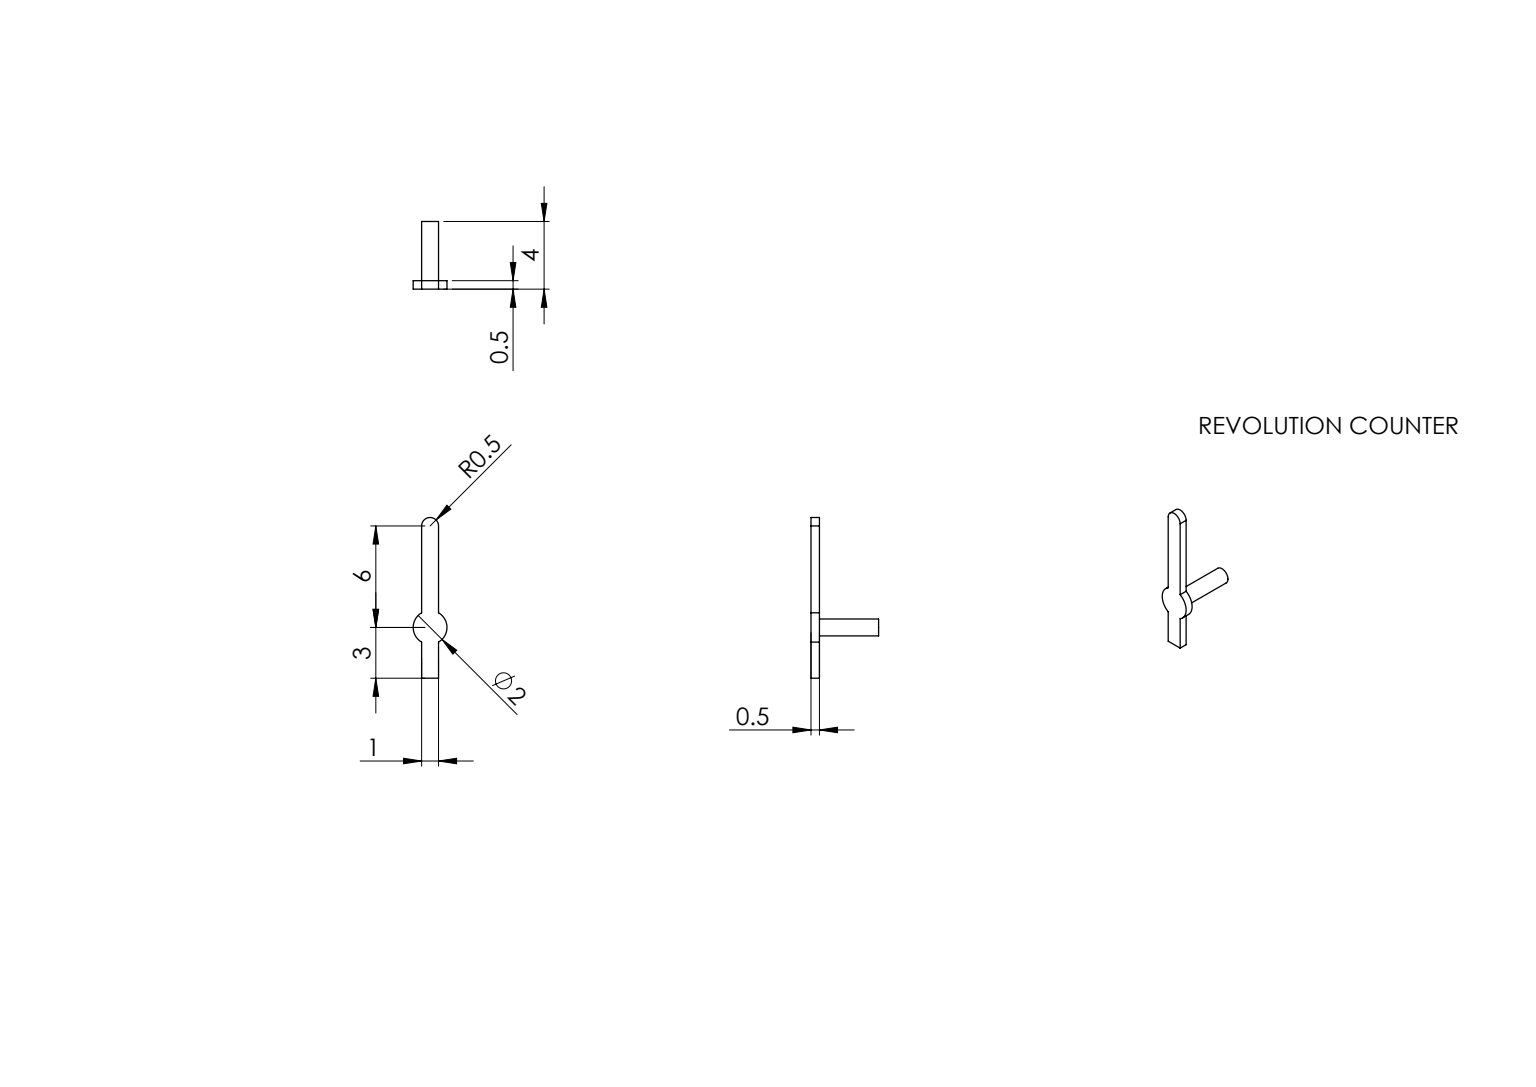
ISO-10303-21;
HEADER;
FILE_DESCRIPTION (('STEP AP214'),
    '1' );
FILE_NAME ('revolution counter.step',
    '2026-10-26T12:50:16',
    ( '' ),
    ( '' ),
    'SwSTEP 2.0',
    'SolidWorks 2026',
    '' );
FILE_SCHEMA (( 'AUTOMOTIVE_DESIGN' ));
ENDSEC;

DATA;
#137=AXIS2_PLACEMENT_3D ( 'NONE', #2400, #6189, #455 ) ;
#284=VERTEX_POINT ( 'NONE', #18909 ) ;
#335=CARTESIAN_POINT ( 'NONE',  ( 0.000000000000000000, 0.000000000000000000, 20.00000000000000000 ) ) ;
#373=CARTESIAN_POINT ( 'NONE',  ( 0.5000000000000001110, 6.123233995736767268E-17, 19.50000000000000000 ) ) ;
#380=VERTEX_POINT ( 'NONE', #21626 ) ;
#455=DIRECTION ( 'NONE',  ( 1.000000000000000000, 0.000000000000000000, 0.000000000000000000 ) ) ;
#566=DIRECTION ( 'NONE',  ( 0.000000000000000000, 0.000000000000000000, 1.000000000000000000 ) ) ;
#582=( GEOMETRIC_REPRESENTATION_CONTEXT ( 3 ) GLOBAL_UNCERTAINTY_ASSIGNED_CONTEXT ( ( #20915 ) ) GLOBAL_UNIT_ASSIGNED_CONTEXT ( ( #19068, #4949, #20517 ) ) REPRESENTATION_CONTEXT ( 'NONE', 'WORKASPACE' ) );
#828=AXIS2_PLACEMENT_3D ( 'NONE', #14567, #3180, #16661 ) ;
#850=AXIS2_PLACEMENT_3D ( 'NONE', #16943, #22823, #13265 ) ;
#918=CARTESIAN_POINT ( 'NONE',  ( 0.5000000000000000000, -2.999999999999999556, 19.50000000000000000 ) ) ;
#963=PLANE ( 'NONE',  #13721 ) ;
#1144=EDGE_CURVE ( 'NONE', #20048, #24513, #24920, .T. ) ;
#1198=DIRECTION ( 'NONE',  ( 1.000000000000000000, 0.000000000000000000, 0.000000000000000000 ) ) ;
#1235=ORIENTED_EDGE ( 'NONE', *, *, #22619, .T. ) ;
#1238=ADVANCED_FACE ( 'NONE', ( #9863 ), #7774, .T. ) ;
#1249=AXIS2_PLACEMENT_3D ( 'NONE', #11596, #19570, #3891 ) ;
#1274=VECTOR ( 'NONE', #23416, 1000.000000000000000 ) ;
#1303=ADVANCED_BREP_SHAPE_REPRESENTATION ( '', ( #5435, #21036 ), #582 ) ;
#1310=AXIS2_PLACEMENT_3D ( 'NONE', #12384, #20350, #10407 ) ;
#1424=FACE_OUTER_BOUND ( 'NONE', #1773, .T. ) ;
#1576=LINE ( 'NONE', #19611, #1274 ) ;
#1773=EDGE_LOOP ( 'NONE', ( #24159, #22801, #5797, #22926 ) ) ;
#1809=EDGE_CURVE ( 'NONE', #2418, #22249, #8902, .T. ) ;
#1853=CARTESIAN_POINT ( 'NONE',  ( -0.5000000000000000000, 6.000000000000000000, 20.00000000000000000 ) ) ;
#2018=DIRECTION ( 'NONE',  ( -0.000000000000000000, -1.000000000000000000, 0.000000000000000000 ) ) ;
#2037=CIRCLE ( 'NONE', #10361, 0.5000000000000000000 ) ;
#2117=ORIENTED_EDGE ( 'NONE', *, *, #6935, .T. ) ;
#2213=ORIENTED_EDGE ( 'NONE', *, *, #1809, .F. ) ;
#2224=( LENGTH_UNIT ( ) NAMED_UNIT ( * ) SI_UNIT ( .MILLI., .METRE. ) );
#2233=AXIS2_PLACEMENT_3D ( 'NONE', #13758, #15729, #7485 ) ;
#2254=VERTEX_POINT ( 'NONE', #17304 ) ;
#2278=EDGE_CURVE ( 'NONE', #11678, #7709, #7918, .T. ) ;
#2363=ORIENTED_EDGE ( 'NONE', *, *, #13575, .T. ) ;
#2369=ORIENTED_EDGE ( 'NONE', *, *, #6160, .F. ) ;
#2400=CARTESIAN_POINT ( 'NONE',  ( 0.000000000000000000, 0.000000000000000000, 19.50000000000000000 ) ) ;
#2418=VERTEX_POINT ( 'NONE', #14656 ) ;
#2611=VECTOR ( 'NONE', #3149, 1000.000000000000000 ) ;
#2661=STYLED_ITEM ( 'NONE', ( #20909 ), #1303 ) ;
#2797=DIRECTION ( 'NONE',  ( -0.000000000000000000, 0.000000000000000000, 1.000000000000000000 ) ) ;
#2884=ORIENTED_EDGE ( 'NONE', *, *, #22262, .T. ) ;
#2904=AXIS2_PLACEMENT_3D ( 'NONE', #9180, #7226, #15209 ) ;
#2905=DIRECTION ( 'NONE',  ( 0.000000000000000000, 0.000000000000000000, 1.000000000000000000 ) ) ;
#2957=AXIS2_PLACEMENT_3D ( 'NONE', #24182, #8117, #20255 ) ;
#2996=( NAMED_UNIT ( * ) SI_UNIT ( $, .STERADIAN. ) SOLID_ANGLE_UNIT ( ) );
#3029=EDGE_CURVE ( 'NONE', #15016, #11472, #8357, .T. ) ;
#3072=STYLED_ITEM('',(#25900),#5435);
#3121=SURFACE_SIDE_STYLE ('',( #22749 ) ) ;
#3126=UNCERTAINTY_MEASURE_WITH_UNIT (LENGTH_MEASURE( 1.000000000000000082E-05 ), #6522, 'distance_accuracy_value', 'NONE');
#3140=ORIENTED_EDGE ( 'NONE', *, *, #3029, .F. ) ;
#3144=ADVANCED_FACE ( 'NONE', ( #15239 ), #5034, .F. ) ;
#3145=ORIENTED_EDGE ( 'NONE', *, *, #21940, .T. ) ;
#3148=EDGE_LOOP ( 'NONE', ( #22343, #13600, #19888, #25002 ) ) ;
#3149=DIRECTION ( 'NONE',  ( -0.000000000000000000, -1.000000000000000000, 0.000000000000000000 ) ) ;
#3180=DIRECTION ( 'NONE',  ( -0.000000000000000000, -0.000000000000000000, -1.000000000000000000 ) ) ;
#3246=DIRECTION ( 'NONE',  ( 0.000000000000000000, 0.000000000000000000, 1.000000000000000000 ) ) ;
#3285=DIRECTION ( 'NONE',  ( 0.000000000000000000, 0.000000000000000000, 1.000000000000000000 ) ) ;
#3847=VECTOR ( 'NONE', #2018, 1000.000000000000000 ) ;
#3891=DIRECTION ( 'NONE',  ( 1.000000000000000000, 0.000000000000000000, 0.000000000000000000 ) ) ;
#3915=MECHANICAL_DESIGN_GEOMETRIC_PRESENTATION_REPRESENTATION('',(#3072),#10585);
#4021=ORIENTED_EDGE ( 'NONE', *, *, #15996, .F. ) ;
#4113=CARTESIAN_POINT ( 'NONE',  ( 0.5000000000000000000, 0.8660254037844387076, 20.00000000000000000 ) ) ;
#4228=ORIENTED_EDGE ( 'NONE', *, *, #21940, .F. ) ;
#4292=CIRCLE ( 'NONE', #21824, 1.000000000000000000 ) ;
#4309=VECTOR ( 'NONE', #5742, 1000.000000000000000 ) ;
#4360=EDGE_CURVE ( 'NONE', #22434, #380, #13096, .T. ) ;
#4373=PLANE ( 'NONE',  #5511 ) ;
#4395=CARTESIAN_POINT ( 'NONE',  ( 0.000000000000000000, 6.000000000000000000, 19.50000000000000000 ) ) ;
#4453=ORIENTED_EDGE ( 'NONE', *, *, #25200, .F. ) ;
#4592=CIRCLE ( 'NONE', #1249, 1.000000000000000000 ) ;
#4632=AXIS2_PLACEMENT_3D ( 'NONE', #23250, #5093, #9512 ) ;
#4709=AXIS2_PLACEMENT_3D ( 'NONE', #21206, #3285, #1198 ) ;
#4716=DIRECTION ( 'NONE',  ( -1.000000000000000000, 0.000000000000000000, 0.000000000000000000 ) ) ;
#4834=DIRECTION ( 'NONE',  ( 0.000000000000000000, 0.000000000000000000, 1.000000000000000000 ) ) ;
#4949=( NAMED_UNIT ( * ) PLANE_ANGLE_UNIT ( ) SI_UNIT ( $, .RADIAN. ) );
#5025=AXIS2_PLACEMENT_3D ( 'NONE', #16249, #566, #16124 ) ;
#5034=PLANE ( 'NONE',  #850 ) ;
#5051=ADVANCED_FACE ( 'NONE', ( #5679 ), #14322, .T. ) ;
#5057=CIRCLE ( 'NONE', #1310, 0.5000000000000001110 ) ;
#5093=DIRECTION ( 'NONE',  ( 0.000000000000000000, 0.000000000000000000, 1.000000000000000000 ) ) ;
#5133=DIRECTION ( 'NONE',  ( 0.000000000000000000, 0.000000000000000000, -1.000000000000000000 ) ) ;
#5179=ORIENTED_EDGE ( 'NONE', *, *, #11117, .T. ) ;
#5204=ORIENTED_EDGE ( 'NONE', *, *, #10339, .T. ) ;
#5292=EDGE_CURVE ( 'NONE', #16864, #284, #17044, .T. ) ;
#5316=ORIENTED_EDGE ( 'NONE', *, *, #22898, .F. ) ;
#5435=MANIFOLD_SOLID_BREP ( 'Extrude-Thin1', #13391 ) ;
#5507=DIRECTION ( 'NONE',  ( 0.000000000000000000, 0.000000000000000000, 1.000000000000000000 ) ) ;
#5511=AXIS2_PLACEMENT_3D ( 'NONE', #22692, #6338, #2797 ) ;
#5585=VERTEX_POINT ( 'NONE', #22475 ) ;
#5669=ORIENTED_EDGE ( 'NONE', *, *, #10339, .F. ) ;
#5679=FACE_OUTER_BOUND ( 'NONE', #25492, .T. ) ;
#5742=DIRECTION ( 'NONE',  ( -0.000000000000000000, -1.000000000000000000, -0.000000000000000000 ) ) ;
#5785=CYLINDRICAL_SURFACE ( 'NONE', #17629, 1.000000000000000000 ) ;
#5787=EDGE_LOOP ( 'NONE', ( #9592, #8354, #12731, #15077 ) ) ;
#5797=ORIENTED_EDGE ( 'NONE', *, *, #15047, .T. ) ;
#5798=ADVANCED_FACE ( 'NONE', ( #14355 ), #10537, .T. ) ;
#5926=DIRECTION ( 'NONE',  ( 1.000000000000000000, 0.000000000000000000, 0.000000000000000000 ) ) ;
#6106=CARTESIAN_POINT ( 'NONE',  ( -0.5000000000000001110, 0.000000000000000000, 20.00000000000000000 ) ) ;
#6124=ORIENTED_EDGE ( 'NONE', *, *, #2278, .T. ) ;
#6160=EDGE_CURVE ( 'NONE', #380, #2254, #22546, .T. ) ;
#6189=DIRECTION ( 'NONE',  ( 0.000000000000000000, 0.000000000000000000, 1.000000000000000000 ) ) ;
#6338=DIRECTION ( 'NONE',  ( -1.000000000000000000, 0.000000000000000000, -0.000000000000000000 ) ) ;
#6515=VERTEX_POINT ( 'NONE', #15857 ) ;
#6522=( LENGTH_UNIT ( ) NAMED_UNIT ( * ) SI_UNIT ( .MILLI., .METRE. ) );
#6662=DIRECTION ( 'NONE',  ( 1.000000000000000000, 0.000000000000000000, 0.000000000000000000 ) ) ;
#6758=CARTESIAN_POINT ( 'NONE',  ( 0.5000000000000000000, -2.999999999999999556, 19.50000000000000000 ) ) ;
#6890=FACE_BOUND ( 'NONE', #24975, .T. ) ;
#6935=EDGE_CURVE ( 'NONE', #18179, #25045, #16534, .T. ) ;
#7002=EDGE_CURVE ( 'NONE', #5585, #2254, #9190, .T. ) ;
#7027=ORIENTED_EDGE ( 'NONE', *, *, #25200, .T. ) ;
#7205=CARTESIAN_POINT ( 'NONE',  ( 0.5000000000000000000, 0.000000000000000000, 20.00000000000000000 ) ) ;
#7226=DIRECTION ( 'NONE',  ( 0.000000000000000000, 0.000000000000000000, 1.000000000000000000 ) ) ;
#7375=ORIENTED_EDGE ( 'NONE', *, *, #12297, .F. ) ;
#7448=ORIENTED_EDGE ( 'NONE', *, *, #6935, .F. ) ;
#7485=DIRECTION ( 'NONE',  ( 1.000000000000000000, 0.000000000000000000, 0.000000000000000000 ) ) ;
#7570=VECTOR ( 'NONE', #24503, 1000.000000000000000 ) ;
#7689=CARTESIAN_POINT ( 'NONE',  ( 0.5000000000000001110, 6.123233995736767268E-17, 16.00000000000000000 ) ) ;
#7709=VERTEX_POINT ( 'NONE', #13877 ) ;
#7747=VECTOR ( 'NONE', #3246, 1000.000000000000000 ) ;
#7762=EDGE_CURVE ( 'NONE', #18701, #11472, #16218, .T. ) ;
#7767=ORIENTED_EDGE ( 'NONE', *, *, #18911, .F. ) ;
#7774=PLANE ( 'NONE',  #10516 ) ;
#7870=LINE ( 'NONE', #12186, #8778 ) ;
#7918=CIRCLE ( 'NONE', #2904, 0.5000000000000001110 ) ;
#8117=DIRECTION ( 'NONE',  ( 0.000000000000000000, 0.000000000000000000, 1.000000000000000000 ) ) ;
#8162=SHAPE_REPRESENTATION ( 'revolution counter', ( #21036 ), #582 ) ;
#8199=EDGE_CURVE ( 'NONE', #20048, #13450, #4292, .T. ) ;
#8223=ORIENTED_EDGE ( 'NONE', *, *, #18466, .T. ) ;
#8354=ORIENTED_EDGE ( 'NONE', *, *, #19672, .F. ) ;
#8357=CIRCLE ( 'NONE', #22561, 1.000000000000000000 ) ;
#8372=DIRECTION ( 'NONE',  ( -0.000000000000000000, -0.000000000000000000, -1.000000000000000000 ) ) ;
#8398=PRODUCT_DEFINITION_SHAPE ( 'NONE', 'NONE',  #22284 ) ;
#8450=EDGE_CURVE ( 'NONE', #284, #9659, #13897, .T. ) ;
#8469=LINE ( 'NONE', #6758, #13830 ) ;
#8479=LINE ( 'NONE', #16582, #16675 ) ;
#8629=DIRECTION ( 'NONE',  ( 0.000000000000000000, 0.000000000000000000, 1.000000000000000000 ) ) ;
#8679=FACE_OUTER_BOUND ( 'NONE', #13542, .T. ) ;
#8778=VECTOR ( 'NONE', #9960, 1000.000000000000000 ) ;
#8902=LINE ( 'NONE', #13203, #7747 ) ;
#8973=PRODUCT_DEFINITION_FORMATION_WITH_SPECIFIED_SOURCE ( 'ANY', '', #18425, .NOT_KNOWN. ) ;
#9120=AXIS2_PLACEMENT_3D ( 'NONE', #16101, #12416, #6662 ) ;
#9129=DIRECTION ( 'NONE',  ( -1.000000000000000000, 0.000000000000000000, 0.000000000000000000 ) ) ;
#9180=CARTESIAN_POINT ( 'NONE',  ( 0.000000000000000000, 0.000000000000000000, 19.50000000000000000 ) ) ;
#9190=LINE ( 'NONE', #21485, #11772 ) ;
#9272=CYLINDRICAL_SURFACE ( 'NONE', #18007, 0.5000000000000001110 ) ;
#9488=CARTESIAN_POINT ( 'NONE',  ( 0.000000000000000000, 0.000000000000000000, 16.00000000000000000 ) ) ;
#9512=DIRECTION ( 'NONE',  ( 1.000000000000000000, 0.000000000000000000, 0.000000000000000000 ) ) ;
#9514=AXIS2_PLACEMENT_3D ( 'NONE', #16606, #20259, #4834 ) ;
#9540=AXIS2_PLACEMENT_3D ( 'NONE', #15202, #19367, #5133 ) ;
#9568=ORIENTED_EDGE ( 'NONE', *, *, #11117, .F. ) ;
#9592=ORIENTED_EDGE ( 'NONE', *, *, #6160, .T. ) ;
#9604=DIRECTION ( 'NONE',  ( -1.000000000000000000, 0.000000000000000000, 0.000000000000000000 ) ) ;
#9659=VERTEX_POINT ( 'NONE', #23698 ) ;
#9730=EDGE_LOOP ( 'NONE', ( #21499, #20363, #15304, #20579 ) ) ;
#9842=PRODUCT_CONTEXT ( 'NONE', #17136, 'mechanical' ) ;
#9863=FACE_OUTER_BOUND ( 'NONE', #15185, .T. ) ;
#9930=CARTESIAN_POINT ( 'NONE',  ( 1.000000000000000000, 0.000000000000000000, 19.50000000000000000 ) ) ;
#9960=DIRECTION ( 'NONE',  ( 0.000000000000000000, 0.000000000000000000, 1.000000000000000000 ) ) ;
#10107=VECTOR ( 'NONE', #16356, 1000.000000000000000 ) ;
#10233=ORIENTED_EDGE ( 'NONE', *, *, #25420, .T. ) ;
#10248=FACE_OUTER_BOUND ( 'NONE', #14469, .T. ) ;
#10327=VERTEX_POINT ( 'NONE', #7689 ) ;
#10339=EDGE_CURVE ( 'NONE', #7709, #6515, #24026, .T. ) ;
#10361=AXIS2_PLACEMENT_3D ( 'NONE', #20848, #22818, #19240 ) ;
#10370=CARTESIAN_POINT ( 'NONE',  ( -0.5000000000000000000, -2.999999999999999556, 19.50000000000000000 ) ) ;
#10407=DIRECTION ( 'NONE',  ( 1.000000000000000000, 0.000000000000000000, 0.000000000000000000 ) ) ;
#10468=EDGE_CURVE ( 'NONE', #24513, #380, #8469, .T. ) ;
#10478=VECTOR ( 'NONE', #21674, 1000.000000000000000 ) ;
#10507=CARTESIAN_POINT ( 'NONE',  ( 0.5000000000000000000, -2.999999999999999556, 20.00000000000000000 ) ) ;
#10516=AXIS2_PLACEMENT_3D ( 'NONE', #17846, #9604, #15887 ) ;
#10537=CYLINDRICAL_SURFACE ( 'NONE', #18131, 0.5000000000000000000 ) ;
#10585=( GEOMETRIC_REPRESENTATION_CONTEXT ( 3 ) GLOBAL_UNCERTAINTY_ASSIGNED_CONTEXT ( ( #13074 ) ) GLOBAL_UNIT_ASSIGNED_CONTEXT ( ( #2224, #24314, #21702 ) ) REPRESENTATION_CONTEXT ( 'NONE', 'WORKASPACE' ) );
#10595=ORIENTED_EDGE ( 'NONE', *, *, #12297, .T. ) ;
#10683=ORIENTED_EDGE ( 'NONE', *, *, #18911, .T. ) ;
#10754=DIRECTION ( 'NONE',  ( 0.000000000000000000, 1.000000000000000000, 0.000000000000000000 ) ) ;
#10825=FILL_AREA_STYLE ('',( #22618 ) ) ;
#10846=ORIENTED_EDGE ( 'NONE', *, *, #4360, .F. ) ;
#10919=DIRECTION ( 'NONE',  ( -0.000000000000000000, -1.000000000000000000, 0.000000000000000000 ) ) ;
#11017=DIRECTION ( 'NONE',  ( -1.000000000000000000, 0.000000000000000000, -0.000000000000000000 ) ) ;
#11075=LINE ( 'NONE', #15270, #14617 ) ;
#11117=EDGE_CURVE ( 'NONE', #6515, #10327, #5057, .T. ) ;
#11124=LINE ( 'NONE', #9930, #10107 ) ;
#11140=DIRECTION ( 'NONE',  ( -0.000000000000000000, -1.000000000000000000, 0.000000000000000000 ) ) ;
#11159=CARTESIAN_POINT ( 'NONE',  ( 0.5000000000000000000, -0.8660254037844387076, 19.50000000000000000 ) ) ;
#11174=SHAPE_DEFINITION_REPRESENTATION ( #8398, #8162 ) ;
#11212=CYLINDRICAL_SURFACE ( 'NONE', #4632, 1.000000000000000000 ) ;
#11272=EDGE_CURVE ( 'NONE', #10327, #6515, #22168, .T. ) ;
#11296=DIRECTION ( 'NONE',  ( 1.000000000000000000, 0.000000000000000000, 0.000000000000000000 ) ) ;
#11455=DIRECTION ( 'NONE',  ( 0.000000000000000000, 0.000000000000000000, 1.000000000000000000 ) ) ;
#11472=VERTEX_POINT ( 'NONE', #4113 ) ;
#11524=VERTEX_POINT ( 'NONE', #10370 ) ;
#11596=CARTESIAN_POINT ( 'NONE',  ( 0.000000000000000000, 0.000000000000000000, 20.00000000000000000 ) ) ;
#11678=VERTEX_POINT ( 'NONE', #373 ) ;
#11761=ORIENTED_EDGE ( 'NONE', *, *, #11272, .T. ) ;
#11772=VECTOR ( 'NONE', #11140, 1000.000000000000000 ) ;
#11798=VECTOR ( 'NONE', #8629, 1000.000000000000000 ) ;
#12013=PLANE ( 'NONE',  #2957 ) ;
#12140=ORIENTED_EDGE ( 'NONE', *, *, #7002, .T. ) ;
#12178=VECTOR ( 'NONE', #18737, 1000.000000000000000 ) ;
#12186=CARTESIAN_POINT ( 'NONE',  ( -0.5000000000000000000, 6.000000000000000000, 19.50000000000000000 ) ) ;
#12256=CARTESIAN_POINT ( 'NONE',  ( 1.000000000000000000, 0.000000000000000000, 20.00000000000000000 ) ) ;
#12293=PLANE ( 'NONE',  #9514 ) ;
#12296=LINE ( 'NONE', #20001, #23727 ) ;
#12297=EDGE_CURVE ( 'NONE', #13450, #15016, #11124, .T. ) ;
#12384=CARTESIAN_POINT ( 'NONE',  ( 0.000000000000000000, 0.000000000000000000, 16.00000000000000000 ) ) ;
#12416=DIRECTION ( 'NONE',  ( 0.000000000000000000, 0.000000000000000000, 1.000000000000000000 ) ) ;
#12449=ORIENTED_EDGE ( 'NONE', *, *, #5292, .T. ) ;
#12497=DIRECTION ( 'NONE',  ( 0.000000000000000000, 0.000000000000000000, 1.000000000000000000 ) ) ;
#12680=SHAPE_REPRESENTATION_RELATIONSHIP ( 'NONE' , 'NONE' ,  #8162, #1303 ) ;
#12731=ORIENTED_EDGE ( 'NONE', *, *, #18466, .F. ) ;
#12735=CARTESIAN_POINT ( 'NONE',  ( -0.5000000000000000000, 0.000000000000000000, 20.00000000000000000 ) ) ;
#12825=EDGE_CURVE ( 'NONE', #22434, #20048, #21935, .T. ) ;
#12826=EDGE_LOOP ( 'NONE', ( #7767, #2213, #1235, #3145 ) ) ;
#12850=DIRECTION ( 'NONE',  ( -0.000000000000000000, 0.000000000000000000, 1.000000000000000000 ) ) ;
#12863=VECTOR ( 'NONE', #4716, 1000.000000000000000 ) ;
#12930=SURFACE_STYLE_USAGE ( .BOTH. , #3121 ) ;
#12988=CARTESIAN_POINT ( 'NONE',  ( 0.5000000000000000000, 0.000000000000000000, 19.50000000000000000 ) ) ;
#13074=UNCERTAINTY_MEASURE_WITH_UNIT (LENGTH_MEASURE( 1.000000000000000082E-05 ), #2224, 'distance_accuracy_value', 'NONE');
#13096=LINE ( 'NONE', #7205, #2611 ) ;
#13127=CARTESIAN_POINT ( 'NONE',  ( -0.5000000000000000000, 0.000000000000000000, 19.50000000000000000 ) ) ;
#13203=CARTESIAN_POINT ( 'NONE',  ( 0.5000000000000000000, 6.000000000000000000, 19.50000000000000000 ) ) ;
#13223=DIRECTION ( 'NONE',  ( 1.000000000000000000, 0.000000000000000000, 0.000000000000000000 ) ) ;
#13256=LINE ( 'NONE', #15347, #16667 ) ;
#13265=DIRECTION ( 'NONE',  ( 1.000000000000000000, 0.000000000000000000, -0.000000000000000000 ) ) ;
#13353=CARTESIAN_POINT ( 'NONE',  ( 0.000000000000000000, 0.000000000000000000, 0.000000000000000000 ) ) ;
#13391=CLOSED_SHELL ( 'NONE', ( #23377, #5051, #24362, #21588, #23018, #3144, #24892, #1238, #5798, #18036, #23325, #24282, #20502, #18328 ) ) ;
#13450=VERTEX_POINT ( 'NONE', #23045 ) ;
#13542=EDGE_LOOP ( 'NONE', ( #4021, #18849, #5204, #5179 ) ) ;
#13575=EDGE_CURVE ( 'NONE', #13450, #18701, #23381, .T. ) ;
#13600=ORIENTED_EDGE ( 'NONE', *, *, #22898, .T. ) ;
#13694=CARTESIAN_POINT ( 'NONE',  ( 0.5000000000000000000, 6.000000000000000000, 20.00000000000000000 ) ) ;
#13721=AXIS2_PLACEMENT_3D ( 'NONE', #12988, #11017, #12850 ) ;
#13758=CARTESIAN_POINT ( 'NONE',  ( 0.000000000000000000, 0.000000000000000000, 20.00000000000000000 ) ) ;
#13830=VECTOR ( 'NONE', #14743, 1000.000000000000000 ) ;
#13877=CARTESIAN_POINT ( 'NONE',  ( -0.5000000000000001110, 0.000000000000000000, 19.50000000000000000 ) ) ;
#13897=CIRCLE ( 'NONE', #4709, 1.000000000000000000 ) ;
#14207=AXIS2_PLACEMENT_3D ( 'NONE', #23673, #5507, #25512 ) ;
#14322=CYLINDRICAL_SURFACE ( 'NONE', #137, 1.000000000000000000 ) ;
#14354=MECHANICAL_DESIGN_GEOMETRIC_PRESENTATION_REPRESENTATION('',(#2661),#20630);
#14355=FACE_OUTER_BOUND ( 'NONE', #12826, .T. ) ;
#14469=EDGE_LOOP ( 'NONE', ( #25385, #23977, #7027, #21240 ) ) ;
#14567=CARTESIAN_POINT ( 'NONE',  ( 0.000000000000000000, 0.000000000000000000, 20.00000000000000000 ) ) ;
#14593=CARTESIAN_POINT ( 'NONE',  ( -0.5000000000000000000, 0.8660254037844387076, 20.00000000000000000 ) ) ;
#14617=VECTOR ( 'NONE', #16977, 1000.000000000000000 ) ;
#14638=( NAMED_UNIT ( * ) PLANE_ANGLE_UNIT ( ) SI_UNIT ( $, .RADIAN. ) );
#14646=LINE ( 'NONE', #22628, #12863 ) ;
#14656=CARTESIAN_POINT ( 'NONE',  ( 0.5000000000000000000, 6.000000000000000000, 19.50000000000000000 ) ) ;
#14689=CARTESIAN_POINT ( 'NONE',  ( 0.000000000000000000, 0.000000000000000000, 19.50000000000000000 ) ) ;
#14743=DIRECTION ( 'NONE',  ( 0.000000000000000000, 0.000000000000000000, 1.000000000000000000 ) ) ;
#14748=CARTESIAN_POINT ( 'NONE',  ( 0.000000000000000000, 0.000000000000000000, 19.50000000000000000 ) ) ;
#14837=CYLINDRICAL_SURFACE ( 'NONE', #828, 0.5000000000000001110 ) ;
#14873=PLANE ( 'NONE',  #17226 ) ;
#14945=FACE_OUTER_BOUND ( 'NONE', #9730, .T. ) ;
#15016=VERTEX_POINT ( 'NONE', #12256 ) ;
#15047=EDGE_CURVE ( 'NONE', #25045, #284, #13256, .T. ) ;
#15077=ORIENTED_EDGE ( 'NONE', *, *, #10468, .T. ) ;
#15168=FACE_OUTER_BOUND ( 'NONE', #24517, .T. ) ;
#15185=EDGE_LOOP ( 'NONE', ( #22569, #7448, #4228, #12449 ) ) ;
#15202=CARTESIAN_POINT ( 'NONE',  ( 0.5000000000000000000, 0.000000000000000000, 19.50000000000000000 ) ) ;
#15209=DIRECTION ( 'NONE',  ( 1.000000000000000000, 0.000000000000000000, 0.000000000000000000 ) ) ;
#15239=FACE_OUTER_BOUND ( 'NONE', #19737, .T. ) ;
#15270=CARTESIAN_POINT ( 'NONE',  ( -0.5000000000000000000, -0.8660254037844387076, 19.50000000000000000 ) ) ;
#15304=ORIENTED_EDGE ( 'NONE', *, *, #10468, .F. ) ;
#15347=CARTESIAN_POINT ( 'NONE',  ( -0.5000000000000000000, 0.8660254037844387076, 19.50000000000000000 ) ) ;
#15703=DIRECTION ( 'NONE',  ( 0.000000000000000000, 0.000000000000000000, 1.000000000000000000 ) ) ;
#15729=DIRECTION ( 'NONE',  ( 0.000000000000000000, 0.000000000000000000, 1.000000000000000000 ) ) ;
#15857=CARTESIAN_POINT ( 'NONE',  ( -0.5000000000000001110, 0.000000000000000000, 16.00000000000000000 ) ) ;
#15887=DIRECTION ( 'NONE',  ( 0.000000000000000000, 0.000000000000000000, 1.000000000000000000 ) ) ;
#15925=AXIS2_PLACEMENT_3D ( 'NONE', #9488, #11455, #21265 ) ;
#15926=EDGE_CURVE ( 'NONE', #7709, #11678, #19974, .T. ) ;
#15996=EDGE_CURVE ( 'NONE', #11678, #10327, #12296, .T. ) ;
#16024=CARTESIAN_POINT ( 'NONE',  ( -0.5000000000000000000, 0.000000000000000000, 19.50000000000000000 ) ) ;
#16101=CARTESIAN_POINT ( 'NONE',  ( 0.000000000000000000, 0.000000000000000000, 19.50000000000000000 ) ) ;
#16124=DIRECTION ( 'NONE',  ( 1.000000000000000000, 0.000000000000000000, 0.000000000000000000 ) ) ;
#16218=LINE ( 'NONE', #20380, #11798 ) ;
#16249=CARTESIAN_POINT ( 'NONE',  ( 0.000000000000000000, 6.000000000000000000, 19.50000000000000000 ) ) ;
#16295=DIRECTION ( 'NONE',  ( 0.000000000000000000, 0.000000000000000000, 1.000000000000000000 ) ) ;
#16356=DIRECTION ( 'NONE',  ( 0.000000000000000000, 0.000000000000000000, 1.000000000000000000 ) ) ;
#16534=LINE ( 'NONE', #12735, #12178 ) ;
#16582=CARTESIAN_POINT ( 'NONE',  ( -0.5000000000000000000, -2.999999999999999556, 19.50000000000000000 ) ) ;
#16606=CARTESIAN_POINT ( 'NONE',  ( 0.5000000000000000000, -2.999999999999999556, 19.50000000000000000 ) ) ;
#16661=DIRECTION ( 'NONE',  ( -1.000000000000000000, 0.000000000000000000, 0.000000000000000000 ) ) ;
#16667=VECTOR ( 'NONE', #21107, 1000.000000000000000 ) ;
#16675=VECTOR ( 'NONE', #18665, 1000.000000000000000 ) ;
#16703=FACE_OUTER_BOUND ( 'NONE', #21184, .T. ) ;
#16799=APPLICATION_CONTEXT ( 'automotive_design' ) ;
#16864=VERTEX_POINT ( 'NONE', #20322 ) ;
#16943=CARTESIAN_POINT ( 'NONE',  ( 0.000000000000000000, 0.000000000000000000, 16.00000000000000000 ) ) ;
#16977=DIRECTION ( 'NONE',  ( -0.000000000000000000, -0.000000000000000000, -1.000000000000000000 ) ) ;
#16995=PRODUCT_DEFINITION_CONTEXT ( 'detailed design', #16799, 'design' ) ;
#17044=LINE ( 'NONE', #13127, #4309 ) ;
#17136=APPLICATION_CONTEXT ( 'automotive_design' ) ;
#17226=AXIS2_PLACEMENT_3D ( 'NONE', #14748, #20752, #20625 ) ;
#17239=ORIENTED_EDGE ( 'NONE', *, *, #8199, .F. ) ;
#17304=CARTESIAN_POINT ( 'NONE',  ( -0.5000000000000000000, -2.999999999999999556, 20.00000000000000000 ) ) ;
#17629=AXIS2_PLACEMENT_3D ( 'NONE', #22004, #23973, #5926 ) ;
#17634=CARTESIAN_POINT ( 'NONE',  ( 0.000000000000000000, 0.000000000000000000, 20.00000000000000000 ) ) ;
#17729=EDGE_CURVE ( 'NONE', #5585, #9659, #11075, .T. ) ;
#17809=ORIENTED_EDGE ( 'NONE', *, *, #2278, .F. ) ;
#17846=CARTESIAN_POINT ( 'NONE',  ( -0.5000000000000000000, 0.000000000000000000, 19.50000000000000000 ) ) ;
#18007=AXIS2_PLACEMENT_3D ( 'NONE', #17634, #19573, #9129 ) ;
#18036=ADVANCED_FACE ( 'NONE', ( #18987 ), #23287, .T. ) ;
#18065=VECTOR ( 'NONE', #10919, 1000.000000000000000 ) ;
#18123=LINE ( 'NONE', #16024, #3847 ) ;
#18131=AXIS2_PLACEMENT_3D ( 'NONE', #4395, #12497, #24527 ) ;
#18179=VERTEX_POINT ( 'NONE', #1853 ) ;
#18224=ORIENTED_EDGE ( 'NONE', *, *, #7762, .T. ) ;
#18328=ADVANCED_FACE ( 'NONE', ( #20379 ), #12293, .F. ) ;
#18425=PRODUCT ( 'revolution counter', 'revolution counter', '', ( #9842 ) ) ;
#18466=EDGE_CURVE ( 'NONE', #24513, #11524, #14646, .T. ) ;
#18665=DIRECTION ( 'NONE',  ( 0.000000000000000000, 0.000000000000000000, 1.000000000000000000 ) ) ;
#18701=VERTEX_POINT ( 'NONE', #21551 ) ;
#18737=DIRECTION ( 'NONE',  ( -0.000000000000000000, -1.000000000000000000, -0.000000000000000000 ) ) ;
#18849=ORIENTED_EDGE ( 'NONE', *, *, #15926, .F. ) ;
#18909=CARTESIAN_POINT ( 'NONE',  ( -0.5000000000000000000, 0.8660254037844387076, 19.50000000000000000 ) ) ;
#18911=EDGE_CURVE ( 'NONE', #22249, #18179, #2037, .T. ) ;
#18987=FACE_OUTER_BOUND ( 'NONE', #3148, .T. ) ;
#18997=ORIENTED_EDGE ( 'NONE', *, *, #5292, .F. ) ;
#19068=( LENGTH_UNIT ( ) NAMED_UNIT ( * ) SI_UNIT ( .MILLI., .METRE. ) );
#19087=ORIENTED_EDGE ( 'NONE', *, *, #15996, .T. ) ;
#19240=DIRECTION ( 'NONE',  ( 1.000000000000000000, 0.000000000000000000, 0.000000000000000000 ) ) ;
#19367=DIRECTION ( 'NONE',  ( 1.000000000000000000, 0.000000000000000000, 0.000000000000000000 ) ) ;
#19380=ORIENTED_EDGE ( 'NONE', *, *, #22619, .F. ) ;
#19570=DIRECTION ( 'NONE',  ( 0.000000000000000000, 0.000000000000000000, 1.000000000000000000 ) ) ;
#19573=DIRECTION ( 'NONE',  ( -0.000000000000000000, -0.000000000000000000, -1.000000000000000000 ) ) ;
#19611=CARTESIAN_POINT ( 'NONE',  ( 0.5000000000000000000, 0.000000000000000000, 19.50000000000000000 ) ) ;
#19672=EDGE_CURVE ( 'NONE', #11524, #2254, #8479, .T. ) ;
#19737=EDGE_LOOP ( 'NONE', ( #9568, #24171 ) ) ;
#19888=ORIENTED_EDGE ( 'NONE', *, *, #1809, .T. ) ;
#19974=CIRCLE ( 'NONE', #9120, 0.5000000000000001110 ) ;
#20001=CARTESIAN_POINT ( 'NONE',  ( 0.5000000000000001110, 6.123233995736767268E-17, 20.00000000000000000 ) ) ;
#20048=VERTEX_POINT ( 'NONE', #11159 ) ;
#20082=ORIENTED_EDGE ( 'NONE', *, *, #25288, .T. ) ;
#20092=CARTESIAN_POINT ( 'NONE',  ( 0.5000000000000000000, -0.8660254037844387076, 19.50000000000000000 ) ) ;
#20185=CARTESIAN_POINT ( 'NONE',  ( 0.5000000000000000000, 0.000000000000000000, 20.00000000000000000 ) ) ;
#20255=DIRECTION ( 'NONE',  ( 1.000000000000000000, 0.000000000000000000, -0.000000000000000000 ) ) ;
#20259=DIRECTION ( 'NONE',  ( 0.000000000000000000, 1.000000000000000000, -0.000000000000000000 ) ) ;
#20299=ORIENTED_EDGE ( 'NONE', *, *, #8450, .F. ) ;
#20322=CARTESIAN_POINT ( 'NONE',  ( -0.5000000000000000000, 6.000000000000000000, 19.50000000000000000 ) ) ;
#20350=DIRECTION ( 'NONE',  ( 0.000000000000000000, 0.000000000000000000, 1.000000000000000000 ) ) ;
#20363=ORIENTED_EDGE ( 'NONE', *, *, #4360, .T. ) ;
#20365=EDGE_LOOP ( 'NONE', ( #7375, #2363, #18224, #3140 ) ) ;
#20379=FACE_OUTER_BOUND ( 'NONE', #5787, .T. ) ;
#20380=CARTESIAN_POINT ( 'NONE',  ( 0.5000000000000000000, 0.8660254037844387076, 19.50000000000000000 ) ) ;
#20502=ADVANCED_FACE ( 'NONE', ( #14945 ), #963, .F. ) ;
#20517=( NAMED_UNIT ( * ) SI_UNIT ( $, .STERADIAN. ) SOLID_ANGLE_UNIT ( ) );
#20579=ORIENTED_EDGE ( 'NONE', *, *, #1144, .F. ) ;
#20609=CARTESIAN_POINT ( 'NONE',  ( 0.5000000000000000000, 0.000000000000000000, 19.50000000000000000 ) ) ;
#20625=DIRECTION ( 'NONE',  ( 1.000000000000000000, 0.000000000000000000, -0.000000000000000000 ) ) ;
#20630=( GEOMETRIC_REPRESENTATION_CONTEXT ( 3 ) GLOBAL_UNCERTAINTY_ASSIGNED_CONTEXT ( ( #3126 ) ) GLOBAL_UNIT_ASSIGNED_CONTEXT ( ( #6522, #14638, #2996 ) ) REPRESENTATION_CONTEXT ( 'NONE', 'WORKASPACE' ) );
#20752=DIRECTION ( 'NONE',  ( 0.000000000000000000, 0.000000000000000000, 1.000000000000000000 ) ) ;
#20848=CARTESIAN_POINT ( 'NONE',  ( 0.000000000000000000, 6.000000000000000000, 20.00000000000000000 ) ) ;
#20909=PRESENTATION_STYLE_ASSIGNMENT (( #12930 ) ) ;
#20915=UNCERTAINTY_MEASURE_WITH_UNIT (LENGTH_MEASURE( 1.000000000000000082E-05 ), #19068, 'distance_accuracy_value', 'NONE');
#21036=AXIS2_PLACEMENT_3D ( 'NONE', #13353, #15703, #13223 ) ;
#21107=DIRECTION ( 'NONE',  ( -0.000000000000000000, -0.000000000000000000, -1.000000000000000000 ) ) ;
#21182=ORIENTED_EDGE ( 'NONE', *, *, #15926, .T. ) ;
#21184=EDGE_LOOP ( 'NONE', ( #17239, #25387, #8223, #4453, #20299, #18997, #19380, #5316, #23090 ) ) ;
#21206=CARTESIAN_POINT ( 'NONE',  ( 0.000000000000000000, 0.000000000000000000, 19.50000000000000000 ) ) ;
#21240=ORIENTED_EDGE ( 'NONE', *, *, #19672, .T. ) ;
#21265=DIRECTION ( 'NONE',  ( 1.000000000000000000, 0.000000000000000000, 0.000000000000000000 ) ) ;
#21485=CARTESIAN_POINT ( 'NONE',  ( -0.5000000000000000000, 0.000000000000000000, 20.00000000000000000 ) ) ;
#21497=FACE_OUTER_BOUND ( 'NONE', #20365, .T. ) ;
#21499=ORIENTED_EDGE ( 'NONE', *, *, #12825, .F. ) ;
#21551=CARTESIAN_POINT ( 'NONE',  ( 0.5000000000000000000, 0.8660254037844387076, 19.50000000000000000 ) ) ;
#21588=ADVANCED_FACE ( 'NONE', ( #8679 ), #14837, .T. ) ;
#21626=CARTESIAN_POINT ( 'NONE',  ( 0.5000000000000000000, -2.999999999999999556, 20.00000000000000000 ) ) ;
#21674=DIRECTION ( 'NONE',  ( -0.000000000000000000, -0.000000000000000000, -1.000000000000000000 ) ) ;
#21702=( NAMED_UNIT ( * ) SI_UNIT ( $, .STERADIAN. ) SOLID_ANGLE_UNIT ( ) );
#21824=AXIS2_PLACEMENT_3D ( 'NONE', #14689, #2905, #24118 ) ;
#21935=LINE ( 'NONE', #20092, #22227 ) ;
#21940=EDGE_CURVE ( 'NONE', #16864, #18179, #7870, .T. ) ;
#22004=CARTESIAN_POINT ( 'NONE',  ( 0.000000000000000000, 0.000000000000000000, 19.50000000000000000 ) ) ;
#22088=FACE_OUTER_BOUND ( 'NONE', #23915, .T. ) ;
#22168=CIRCLE ( 'NONE', #15925, 0.5000000000000001110 ) ;
#22227=VECTOR ( 'NONE', #23900, 1000.000000000000000 ) ;
#22249=VERTEX_POINT ( 'NONE', #13694 ) ;
#22258=VECTOR ( 'NONE', #10754, 1000.000000000000000 ) ;
#22262=EDGE_CURVE ( 'NONE', #22434, #15016, #4592, .T. ) ;
#22277=COLOUR_RGB ( '',0.8941176470588234615, 0.8941176470588234615, 0.8941176470588234615 ) ;
#22283=ORIENTED_EDGE ( 'NONE', *, *, #12825, .T. ) ;
#22284=PRODUCT_DEFINITION ( 'UNKNOWN', '', #8973, #16995 ) ;
#22302=ORIENTED_EDGE ( 'NONE', *, *, #22262, .F. ) ;
#22343=ORIENTED_EDGE ( 'NONE', *, *, #7762, .F. ) ;
#22408=LINE ( 'NONE', #20185, #22258 ) ;
#22434=VERTEX_POINT ( 'NONE', #23218 ) ;
#22475=CARTESIAN_POINT ( 'NONE',  ( -0.5000000000000000000, -0.8660254037844387076, 20.00000000000000000 ) ) ;
#22546=LINE ( 'NONE', #10507, #7570 ) ;
#22561=AXIS2_PLACEMENT_3D ( 'NONE', #335, #16295, #11296 ) ;
#22569=ORIENTED_EDGE ( 'NONE', *, *, #15047, .F. ) ;
#22578=CIRCLE ( 'NONE', #5025, 0.5000000000000000000 ) ;
#22618=FILL_AREA_STYLE_COLOUR ( '', #22277 ) ;
#22619=EDGE_CURVE ( 'NONE', #2418, #16864, #22578, .T. ) ;
#22628=CARTESIAN_POINT ( 'NONE',  ( 0.5000000000000000000, -2.999999999999999556, 19.50000000000000000 ) ) ;
#22692=CARTESIAN_POINT ( 'NONE',  ( -0.5000000000000000000, 0.000000000000000000, 19.50000000000000000 ) ) ;
#22749=SURFACE_STYLE_FILL_AREA ( #10825 ) ;
#22801=ORIENTED_EDGE ( 'NONE', *, *, #25420, .F. ) ;
#22818=DIRECTION ( 'NONE',  ( 0.000000000000000000, 0.000000000000000000, 1.000000000000000000 ) ) ;
#22823=DIRECTION ( 'NONE',  ( 0.000000000000000000, 0.000000000000000000, 1.000000000000000000 ) ) ;
#22898=EDGE_CURVE ( 'NONE', #18701, #2418, #1576, .T. ) ;
#22926=ORIENTED_EDGE ( 'NONE', *, *, #8450, .T. ) ;
#23018=ADVANCED_FACE ( 'NONE', ( #22088 ), #12013, .T. ) ;
#23045=CARTESIAN_POINT ( 'NONE',  ( 1.000000000000000000, 0.000000000000000000, 19.50000000000000000 ) ) ;
#23090=ORIENTED_EDGE ( 'NONE', *, *, #13575, .F. ) ;
#23218=CARTESIAN_POINT ( 'NONE',  ( 0.5000000000000000000, -0.8660254037844387076, 20.00000000000000000 ) ) ;
#23250=CARTESIAN_POINT ( 'NONE',  ( 0.000000000000000000, 0.000000000000000000, 19.50000000000000000 ) ) ;
#23287=PLANE ( 'NONE',  #9540 ) ;
#23325=ADVANCED_FACE ( 'NONE', ( #1424 ), #11212, .T. ) ;
#23377=ADVANCED_FACE ( 'NONE', ( #15168 ), #9272, .T. ) ;
#23381=CIRCLE ( 'NONE', #14207, 1.000000000000000000 ) ;
#23416=DIRECTION ( 'NONE',  ( 0.000000000000000000, 1.000000000000000000, 0.000000000000000000 ) ) ;
#23673=CARTESIAN_POINT ( 'NONE',  ( 0.000000000000000000, 0.000000000000000000, 19.50000000000000000 ) ) ;
#23698=CARTESIAN_POINT ( 'NONE',  ( -0.5000000000000000000, -0.8660254037844387076, 19.50000000000000000 ) ) ;
#23727=VECTOR ( 'NONE', #8372, 1000.000000000000000 ) ;
#23900=DIRECTION ( 'NONE',  ( -0.000000000000000000, -0.000000000000000000, -1.000000000000000000 ) ) ;
#23915=EDGE_LOOP ( 'NONE', ( #10233, #12140, #2369, #10846, #2884, #25494, #20082, #10683, #2117 ) ) ;
#23973=DIRECTION ( 'NONE',  ( 0.000000000000000000, 0.000000000000000000, 1.000000000000000000 ) ) ;
#23977=ORIENTED_EDGE ( 'NONE', *, *, #17729, .T. ) ;
#24026=LINE ( 'NONE', #6106, #10478 ) ;
#24118=DIRECTION ( 'NONE',  ( 1.000000000000000000, 0.000000000000000000, 0.000000000000000000 ) ) ;
#24159=ORIENTED_EDGE ( 'NONE', *, *, #17729, .F. ) ;
#24171=ORIENTED_EDGE ( 'NONE', *, *, #11272, .F. ) ;
#24182=CARTESIAN_POINT ( 'NONE',  ( 0.000000000000000000, 0.000000000000000000, 20.00000000000000000 ) ) ;
#24282=ADVANCED_FACE ( 'NONE', ( #10248 ), #4373, .T. ) ;
#24314=( NAMED_UNIT ( * ) PLANE_ANGLE_UNIT ( ) SI_UNIT ( $, .RADIAN. ) );
#24351=CIRCLE ( 'NONE', #2233, 1.000000000000000000 ) ;
#24362=ADVANCED_FACE ( 'NONE', ( #21497 ), #5785, .T. ) ;
#24503=DIRECTION ( 'NONE',  ( -1.000000000000000000, 0.000000000000000000, 0.000000000000000000 ) ) ;
#24513=VERTEX_POINT ( 'NONE', #918 ) ;
#24517=EDGE_LOOP ( 'NONE', ( #17809, #19087, #11761, #5669 ) ) ;
#24527=DIRECTION ( 'NONE',  ( 1.000000000000000000, 0.000000000000000000, 0.000000000000000000 ) ) ;
#24892=ADVANCED_FACE ( 'NONE', ( #16703, #6890 ), #14873, .F. ) ;
#24920=LINE ( 'NONE', #20609, #18065 ) ;
#24975=EDGE_LOOP ( 'NONE', ( #21182, #6124 ) ) ;
#25002=ORIENTED_EDGE ( 'NONE', *, *, #25288, .F. ) ;
#25045=VERTEX_POINT ( 'NONE', #14593 ) ;
#25111=ORIENTED_EDGE ( 'NONE', *, *, #8199, .T. ) ;
#25200=EDGE_CURVE ( 'NONE', #9659, #11524, #18123, .T. ) ;
#25288=EDGE_CURVE ( 'NONE', #11472, #22249, #22408, .T. ) ;
#25385=ORIENTED_EDGE ( 'NONE', *, *, #7002, .F. ) ;
#25387=ORIENTED_EDGE ( 'NONE', *, *, #1144, .T. ) ;
#25420=EDGE_CURVE ( 'NONE', #25045, #5585, #24351, .T. ) ;
#25492=EDGE_LOOP ( 'NONE', ( #25111, #10595, #22302, #22283 ) ) ;
#25494=ORIENTED_EDGE ( 'NONE', *, *, #3029, .T. ) ;
#25512=DIRECTION ( 'NONE',  ( 1.000000000000000000, 0.000000000000000000, 0.000000000000000000 ) ) ;
#25894=COLOUR_RGB('Light Blue',0.38,0.62,0.78);
#25895=FILL_AREA_STYLE_COLOUR('',#25894);
#25896=FILL_AREA_STYLE('',(#25895));
#25897=SURFACE_STYLE_FILL_AREA(#25896);
#25898=SURFACE_SIDE_STYLE('',(#25897));
#25899=SURFACE_STYLE_USAGE(.BOTH.,#25898);
#25900=PRESENTATION_STYLE_ASSIGNMENT((#25899));
ENDSEC;
END-ISO-10303-21;
